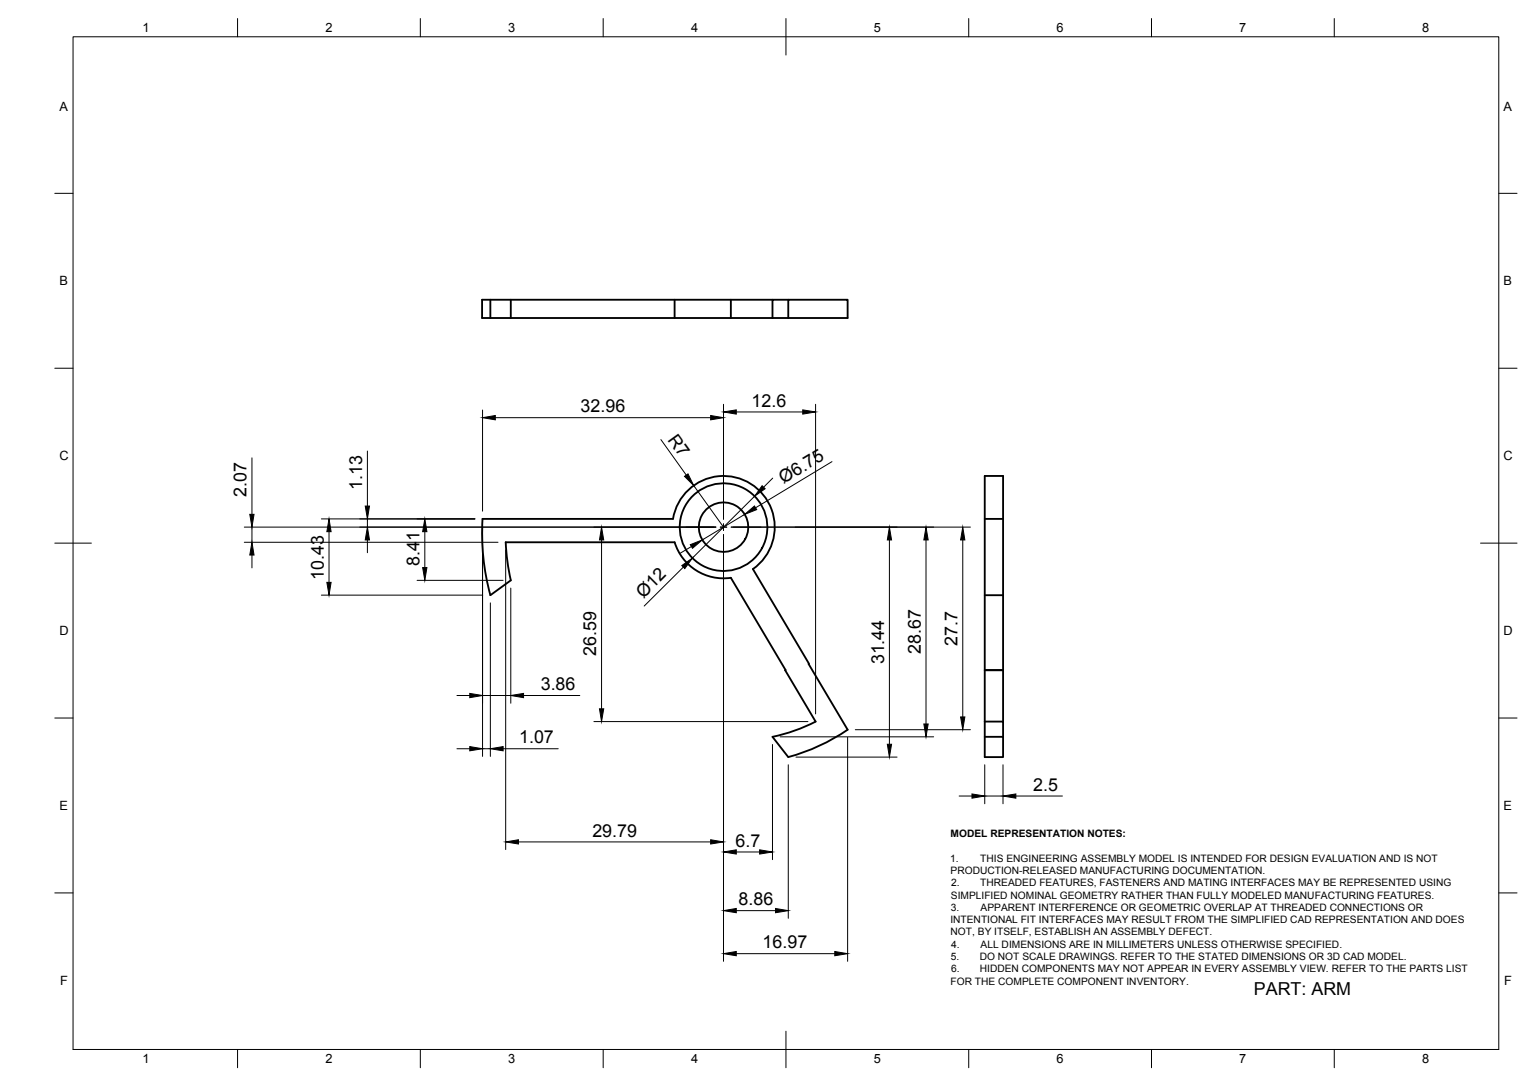
ISO-10303-21;
HEADER;
/* Generated by software containing ST-Developer
 * from STEP Tools, Inc. (www.steptools.com) 
 */

FILE_DESCRIPTION(
/* description */ (''),
/* implementation_level */ '2;1');

FILE_NAME(
/* name */ 'Arm.step',
/* time_stamp */ '2026-10-04T15:18:51-07:00',
/* author */ (''),
/* organization */ (''),
/* preprocessor_version */ 'ST-DEVELOPER v20.2',
/* originating_system */ 'Autodesk Translation Framework v15.15.0.0',
/* authorisation */ '');

FILE_SCHEMA (('AUTOMOTIVE_DESIGN { 1 0 10303 214 3 1 1 }'));
ENDSEC;

DATA;
#10=MECHANICAL_DESIGN_GEOMETRIC_PRESENTATION_REPRESENTATION('',(#77),#9891);
#58=SHAPE_REPRESENTATION_RELATIONSHIP('SRR','None',#9929,#66);
#66=ADVANCED_BREP_SHAPE_REPRESENTATION('',(#91),#9889);
#77=STYLED_ITEM('',(#9975),#91);
#91=MANIFOLD_SOLID_BREP('Body1',#5625);
#140=FACE_BOUND('',#1032,.T.);
#141=FACE_BOUND('',#1034,.T.);
#142=FACE_BOUND('',#1042,.T.);
#306=PLANE('',#6186);
#307=PLANE('',#6188);
#308=PLANE('',#6195);
#309=PLANE('',#6198);
#310=PLANE('',#6201);
#311=PLANE('',#6202);
#312=PLANE('',#6203);
#313=PLANE('',#6209);
#314=PLANE('',#6210);
#315=PLANE('',#6213);
#316=PLANE('',#6215);
#317=PLANE('',#6217);
#318=PLANE('',#6219);
#656=FACE_OUTER_BOUND('',#1030,.T.);
#657=FACE_OUTER_BOUND('',#1031,.T.);
#658=FACE_OUTER_BOUND('',#1033,.T.);
#659=FACE_OUTER_BOUND('',#1035,.T.);
#660=FACE_OUTER_BOUND('',#1036,.T.);
#661=FACE_OUTER_BOUND('',#1037,.T.);
#662=FACE_OUTER_BOUND('',#1038,.T.);
#663=FACE_OUTER_BOUND('',#1039,.T.);
#664=FACE_OUTER_BOUND('',#1040,.T.);
#665=FACE_OUTER_BOUND('',#1041,.T.);
#666=FACE_OUTER_BOUND('',#1043,.T.);
#667=FACE_OUTER_BOUND('',#1044,.T.);
#668=FACE_OUTER_BOUND('',#1045,.T.);
#669=FACE_OUTER_BOUND('',#1046,.T.);
#670=FACE_OUTER_BOUND('',#1047,.T.);
#671=FACE_OUTER_BOUND('',#1048,.T.);
#672=FACE_OUTER_BOUND('',#1049,.T.);
#673=FACE_OUTER_BOUND('',#1050,.T.);
#674=FACE_OUTER_BOUND('',#1051,.T.);
#675=FACE_OUTER_BOUND('',#1052,.T.);
#676=FACE_OUTER_BOUND('',#1053,.T.);
#1030=EDGE_LOOP('',(#4886,#4887,#4888,#4889));
#1031=EDGE_LOOP('',(#4890));
#1032=EDGE_LOOP('',(#4891));
#1033=EDGE_LOOP('',(#4892,#4893,#4894,#4895,#4896,#4897,#4898,#4899,#4900,
#4901,#4902,#4903,#4904,#4905,#4906,#4907));
#1034=EDGE_LOOP('',(#4908));
#1035=EDGE_LOOP('',(#4909,#4910,#4911,#4912));
#1036=EDGE_LOOP('',(#4913,#4914,#4915,#4916));
#1037=EDGE_LOOP('',(#4917,#4918,#4919,#4920));
#1038=EDGE_LOOP('',(#4921,#4922,#4923,#4924));
#1039=EDGE_LOOP('',(#4925,#4926,#4927,#4928));
#1040=EDGE_LOOP('',(#4929,#4930,#4931,#4932));
#1041=EDGE_LOOP('',(#4933,#4934,#4935,#4936,#4937,#4938,#4939,#4940,#4941,
#4942,#4943,#4944,#4945,#4946,#4947,#4948));
#1042=EDGE_LOOP('',(#4949));
#1043=EDGE_LOOP('',(#4950,#4951,#4952,#4953));
#1044=EDGE_LOOP('',(#4954,#4955,#4956,#4957));
#1045=EDGE_LOOP('',(#4958,#4959,#4960,#4961));
#1046=EDGE_LOOP('',(#4962,#4963,#4964,#4965));
#1047=EDGE_LOOP('',(#4966,#4967,#4968,#4969));
#1048=EDGE_LOOP('',(#4970,#4971,#4972,#4973));
#1049=EDGE_LOOP('',(#4974,#4975,#4976,#4977));
#1050=EDGE_LOOP('',(#4978,#4979,#4980,#4981));
#1051=EDGE_LOOP('',(#4982,#4983,#4984,#4985));
#1052=EDGE_LOOP('',(#4986,#4987,#4988,#4989));
#1053=EDGE_LOOP('',(#4990,#4991,#4992,#4993));
#1536=LINE('',#9530,#2000);
#1537=LINE('',#9538,#2001);
#1538=LINE('',#9540,#2002);
#1539=LINE('',#9542,#2003);
#1540=LINE('',#9546,#2004);
#1541=LINE('',#9550,#2005);
#1542=LINE('',#9554,#2006);
#1543=LINE('',#9558,#2007);
#1544=LINE('',#9560,#2008);
#1545=LINE('',#9562,#2009);
#1546=LINE('',#9566,#2010);
#1547=LINE('',#9570,#2011);
#1548=LINE('',#9572,#2012);
#1549=LINE('',#9573,#2013);
#1550=LINE('',#9578,#2014);
#1551=LINE('',#9579,#2015);
#1552=LINE('',#9582,#2016);
#1553=LINE('',#9583,#2017);
#1554=LINE('',#9587,#2018);
#1555=LINE('',#9590,#2019);
#1556=LINE('',#9591,#2020);
#1557=LINE('',#9593,#2021);
#1558=LINE('',#9596,#2022);
#1559=LINE('',#9598,#2023);
#1560=LINE('',#9602,#2024);
#1561=LINE('',#9606,#2025);
#1562=LINE('',#9610,#2026);
#1563=LINE('',#9613,#2027);
#1564=LINE('',#9617,#2028);
#1565=LINE('',#9619,#2029);
#1566=LINE('',#9621,#2030);
#1567=LINE('',#9623,#2031);
#1568=LINE('',#9625,#2032);
#1569=LINE('',#9627,#2033);
#1570=LINE('',#9629,#2034);
#1571=LINE('',#9631,#2035);
#1572=LINE('',#9633,#2036);
#1573=LINE('',#9635,#2037);
#2000=VECTOR('',#7707,3.37715398312954);
#2001=VECTOR('',#7716,10.);
#2002=VECTOR('',#7717,10.);
#2003=VECTOR('',#7718,10.);
#2004=VECTOR('',#7721,10.);
#2005=VECTOR('',#7724,10.);
#2006=VECTOR('',#7727,10.);
#2007=VECTOR('',#7730,10.);
#2008=VECTOR('',#7731,10.);
#2009=VECTOR('',#7732,10.);
#2010=VECTOR('',#7735,10.);
#2011=VECTOR('',#7740,10.);
#2012=VECTOR('',#7741,10.);
#2013=VECTOR('',#7742,9.99999999999999);
#2014=VECTOR('',#7747,10.);
#2015=VECTOR('',#7748,10.);
#2016=VECTOR('',#7751,10.);
#2017=VECTOR('',#7752,10.);
#2018=VECTOR('',#7757,10.);
#2019=VECTOR('',#7760,10.);
#2020=VECTOR('',#7761,10.);
#2021=VECTOR('',#7764,10.);
#2022=VECTOR('',#7767,9.99999999999999);
#2023=VECTOR('',#7768,10.);
#2024=VECTOR('',#7771,10.);
#2025=VECTOR('',#7774,10.);
#2026=VECTOR('',#7777,10.);
#2027=VECTOR('',#7780,10.);
#2028=VECTOR('',#7785,10.);
#2029=VECTOR('',#7788,10.);
#2030=VECTOR('',#7791,6.00000000000001);
#2031=VECTOR('',#7794,10.);
#2032=VECTOR('',#7797,10.);
#2033=VECTOR('',#7800,10.);
#2034=VECTOR('',#7803,10.);
#2035=VECTOR('',#7806,10.);
#2036=VECTOR('',#7809,10.);
#2037=VECTOR('',#7812,10.);
#2267=CIRCLE('',#6184,3.37715398312954);
#2268=CIRCLE('',#6185,3.37715398312954);
#2269=CIRCLE('',#6187,6.00000000000001);
#2270=CIRCLE('',#6189,7.00000000000001);
#2271=CIRCLE('',#6190,29.0155772121002);
#2272=CIRCLE('',#6191,32.2155772121002);
#2273=CIRCLE('',#6192,7.00000000000001);
#2274=CIRCLE('',#6193,26.714151341222);
#2275=CIRCLE('',#6194,23.514151341222);
#2276=CIRCLE('',#6197,26.714151341222);
#2277=CIRCLE('',#6200,23.514151341222);
#2278=CIRCLE('',#6204,7.00000000000001);
#2279=CIRCLE('',#6205,32.2155772121003);
#2280=CIRCLE('',#6206,29.0155772121003);
#2281=CIRCLE('',#6207,7.00000000000001);
#2282=CIRCLE('',#6208,6.00000000000001);
#2770=VERTEX_POINT('',#9527);
#2771=VERTEX_POINT('',#9529);
#2772=VERTEX_POINT('',#9533);
#2773=VERTEX_POINT('',#9536);
#2774=VERTEX_POINT('',#9537);
#2775=VERTEX_POINT('',#9539);
#2776=VERTEX_POINT('',#9541);
#2777=VERTEX_POINT('',#9543);
#2778=VERTEX_POINT('',#9545);
#2779=VERTEX_POINT('',#9547);
#2780=VERTEX_POINT('',#9549);
#2781=VERTEX_POINT('',#9551);
#2782=VERTEX_POINT('',#9553);
#2783=VERTEX_POINT('',#9555);
#2784=VERTEX_POINT('',#9557);
#2785=VERTEX_POINT('',#9559);
#2786=VERTEX_POINT('',#9561);
#2787=VERTEX_POINT('',#9563);
#2788=VERTEX_POINT('',#9565);
#2789=VERTEX_POINT('',#9569);
#2790=VERTEX_POINT('',#9571);
#2791=VERTEX_POINT('',#9575);
#2792=VERTEX_POINT('',#9576);
#2793=VERTEX_POINT('',#9581);
#2794=VERTEX_POINT('',#9585);
#2795=VERTEX_POINT('',#9589);
#2796=VERTEX_POINT('',#9595);
#2797=VERTEX_POINT('',#9597);
#2798=VERTEX_POINT('',#9599);
#2799=VERTEX_POINT('',#9601);
#2800=VERTEX_POINT('',#9603);
#2801=VERTEX_POINT('',#9605);
#2802=VERTEX_POINT('',#9607);
#2803=VERTEX_POINT('',#9609);
#2804=VERTEX_POINT('',#9611);
#2805=VERTEX_POINT('',#9614);
#3488=EDGE_CURVE('',#2770,#2770,#2267,.F.);
#3489=EDGE_CURVE('',#2770,#2771,#1536,.T.);
#3490=EDGE_CURVE('',#2771,#2771,#2268,.T.);
#3491=EDGE_CURVE('',#2772,#2772,#2269,.T.);
#3492=EDGE_CURVE('',#2773,#2774,#1537,.T.);
#3493=EDGE_CURVE('',#2774,#2775,#1538,.T.);
#3494=EDGE_CURVE('',#2775,#2776,#1539,.T.);
#3495=EDGE_CURVE('',#2776,#2777,#2270,.T.);
#3496=EDGE_CURVE('',#2777,#2778,#1540,.T.);
#3497=EDGE_CURVE('',#2778,#2779,#2271,.T.);
#3498=EDGE_CURVE('',#2779,#2780,#1541,.T.);
#3499=EDGE_CURVE('',#2780,#2781,#2272,.T.);
#3500=EDGE_CURVE('',#2781,#2782,#1542,.T.);
#3501=EDGE_CURVE('',#2782,#2783,#2273,.T.);
#3502=EDGE_CURVE('',#2783,#2784,#1543,.T.);
#3503=EDGE_CURVE('',#2784,#2785,#1544,.T.);
#3504=EDGE_CURVE('',#2785,#2786,#1545,.T.);
#3505=EDGE_CURVE('',#2786,#2787,#2274,.T.);
#3506=EDGE_CURVE('',#2787,#2788,#1546,.T.);
#3507=EDGE_CURVE('',#2788,#2773,#2275,.T.);
#3508=EDGE_CURVE('',#2775,#2789,#1547,.T.);
#3509=EDGE_CURVE('',#2774,#2790,#1548,.T.);
#3510=EDGE_CURVE('',#2790,#2789,#1549,.T.);
#3511=EDGE_CURVE('',#2791,#2792,#2276,.T.);
#3512=EDGE_CURVE('',#2792,#2787,#1550,.T.);
#3513=EDGE_CURVE('',#2791,#2786,#1551,.T.);
#3514=EDGE_CURVE('',#2792,#2793,#1552,.T.);
#3515=EDGE_CURVE('',#2793,#2788,#1553,.T.);
#3516=EDGE_CURVE('',#2794,#2793,#2277,.T.);
#3517=EDGE_CURVE('',#2794,#2773,#1554,.T.);
#3518=EDGE_CURVE('',#2795,#2785,#1555,.T.);
#3519=EDGE_CURVE('',#2791,#2795,#1556,.T.);
#3520=EDGE_CURVE('',#2794,#2790,#1557,.T.);
#3521=EDGE_CURVE('',#2795,#2796,#1558,.T.);
#3522=EDGE_CURVE('',#2796,#2797,#1559,.T.);
#3523=EDGE_CURVE('',#2798,#2797,#2278,.T.);
#3524=EDGE_CURVE('',#2798,#2799,#1560,.T.);
#3525=EDGE_CURVE('',#2800,#2799,#2279,.T.);
#3526=EDGE_CURVE('',#2801,#2800,#1561,.T.);
#3527=EDGE_CURVE('',#2801,#2802,#2280,.T.);
#3528=EDGE_CURVE('',#2803,#2802,#1562,.T.);
#3529=EDGE_CURVE('',#2804,#2803,#2281,.T.);
#3530=EDGE_CURVE('',#2789,#2804,#1563,.T.);
#3531=EDGE_CURVE('',#2805,#2805,#2282,.T.);
#3532=EDGE_CURVE('',#2796,#2784,#1564,.T.);
#3533=EDGE_CURVE('',#2797,#2783,#1565,.T.);
#3534=EDGE_CURVE('',#2805,#2772,#1566,.T.);
#3535=EDGE_CURVE('',#2798,#2782,#1567,.T.);
#3536=EDGE_CURVE('',#2799,#2781,#1568,.T.);
#3537=EDGE_CURVE('',#2800,#2780,#1569,.T.);
#3538=EDGE_CURVE('',#2801,#2779,#1570,.T.);
#3539=EDGE_CURVE('',#2802,#2778,#1571,.T.);
#3540=EDGE_CURVE('',#2803,#2777,#1572,.T.);
#3541=EDGE_CURVE('',#2804,#2776,#1573,.T.);
#4886=ORIENTED_EDGE('',*,*,#3488,.F.);
#4887=ORIENTED_EDGE('',*,*,#3489,.T.);
#4888=ORIENTED_EDGE('',*,*,#3490,.F.);
#4889=ORIENTED_EDGE('',*,*,#3489,.F.);
#4890=ORIENTED_EDGE('',*,*,#3491,.T.);
#4891=ORIENTED_EDGE('',*,*,#3488,.T.);
#4892=ORIENTED_EDGE('',*,*,#3492,.T.);
#4893=ORIENTED_EDGE('',*,*,#3493,.T.);
#4894=ORIENTED_EDGE('',*,*,#3494,.T.);
#4895=ORIENTED_EDGE('',*,*,#3495,.T.);
#4896=ORIENTED_EDGE('',*,*,#3496,.T.);
#4897=ORIENTED_EDGE('',*,*,#3497,.T.);
#4898=ORIENTED_EDGE('',*,*,#3498,.T.);
#4899=ORIENTED_EDGE('',*,*,#3499,.T.);
#4900=ORIENTED_EDGE('',*,*,#3500,.T.);
#4901=ORIENTED_EDGE('',*,*,#3501,.T.);
#4902=ORIENTED_EDGE('',*,*,#3502,.T.);
#4903=ORIENTED_EDGE('',*,*,#3503,.T.);
#4904=ORIENTED_EDGE('',*,*,#3504,.T.);
#4905=ORIENTED_EDGE('',*,*,#3505,.T.);
#4906=ORIENTED_EDGE('',*,*,#3506,.T.);
#4907=ORIENTED_EDGE('',*,*,#3507,.T.);
#4908=ORIENTED_EDGE('',*,*,#3490,.T.);
#4909=ORIENTED_EDGE('',*,*,#3508,.F.);
#4910=ORIENTED_EDGE('',*,*,#3493,.F.);
#4911=ORIENTED_EDGE('',*,*,#3509,.T.);
#4912=ORIENTED_EDGE('',*,*,#3510,.T.);
#4913=ORIENTED_EDGE('',*,*,#3511,.T.);
#4914=ORIENTED_EDGE('',*,*,#3512,.T.);
#4915=ORIENTED_EDGE('',*,*,#3505,.F.);
#4916=ORIENTED_EDGE('',*,*,#3513,.F.);
#4917=ORIENTED_EDGE('',*,*,#3514,.T.);
#4918=ORIENTED_EDGE('',*,*,#3515,.T.);
#4919=ORIENTED_EDGE('',*,*,#3506,.F.);
#4920=ORIENTED_EDGE('',*,*,#3512,.F.);
#4921=ORIENTED_EDGE('',*,*,#3516,.F.);
#4922=ORIENTED_EDGE('',*,*,#3517,.T.);
#4923=ORIENTED_EDGE('',*,*,#3507,.F.);
#4924=ORIENTED_EDGE('',*,*,#3515,.F.);
#4925=ORIENTED_EDGE('',*,*,#3518,.F.);
#4926=ORIENTED_EDGE('',*,*,#3519,.F.);
#4927=ORIENTED_EDGE('',*,*,#3513,.T.);
#4928=ORIENTED_EDGE('',*,*,#3504,.F.);
#4929=ORIENTED_EDGE('',*,*,#3509,.F.);
#4930=ORIENTED_EDGE('',*,*,#3492,.F.);
#4931=ORIENTED_EDGE('',*,*,#3517,.F.);
#4932=ORIENTED_EDGE('',*,*,#3520,.T.);
#4933=ORIENTED_EDGE('',*,*,#3510,.F.);
#4934=ORIENTED_EDGE('',*,*,#3520,.F.);
#4935=ORIENTED_EDGE('',*,*,#3516,.T.);
#4936=ORIENTED_EDGE('',*,*,#3514,.F.);
#4937=ORIENTED_EDGE('',*,*,#3511,.F.);
#4938=ORIENTED_EDGE('',*,*,#3519,.T.);
#4939=ORIENTED_EDGE('',*,*,#3521,.T.);
#4940=ORIENTED_EDGE('',*,*,#3522,.T.);
#4941=ORIENTED_EDGE('',*,*,#3523,.F.);
#4942=ORIENTED_EDGE('',*,*,#3524,.T.);
#4943=ORIENTED_EDGE('',*,*,#3525,.F.);
#4944=ORIENTED_EDGE('',*,*,#3526,.F.);
#4945=ORIENTED_EDGE('',*,*,#3527,.T.);
#4946=ORIENTED_EDGE('',*,*,#3528,.F.);
#4947=ORIENTED_EDGE('',*,*,#3529,.F.);
#4948=ORIENTED_EDGE('',*,*,#3530,.F.);
#4949=ORIENTED_EDGE('',*,*,#3531,.F.);
#4950=ORIENTED_EDGE('',*,*,#3518,.T.);
#4951=ORIENTED_EDGE('',*,*,#3503,.F.);
#4952=ORIENTED_EDGE('',*,*,#3532,.F.);
#4953=ORIENTED_EDGE('',*,*,#3521,.F.);
#4954=ORIENTED_EDGE('',*,*,#3532,.T.);
#4955=ORIENTED_EDGE('',*,*,#3502,.F.);
#4956=ORIENTED_EDGE('',*,*,#3533,.F.);
#4957=ORIENTED_EDGE('',*,*,#3522,.F.);
#4958=ORIENTED_EDGE('',*,*,#3531,.T.);
#4959=ORIENTED_EDGE('',*,*,#3534,.T.);
#4960=ORIENTED_EDGE('',*,*,#3491,.F.);
#4961=ORIENTED_EDGE('',*,*,#3534,.F.);
#4962=ORIENTED_EDGE('',*,*,#3523,.T.);
#4963=ORIENTED_EDGE('',*,*,#3533,.T.);
#4964=ORIENTED_EDGE('',*,*,#3501,.F.);
#4965=ORIENTED_EDGE('',*,*,#3535,.F.);
#4966=ORIENTED_EDGE('',*,*,#3524,.F.);
#4967=ORIENTED_EDGE('',*,*,#3535,.T.);
#4968=ORIENTED_EDGE('',*,*,#3500,.F.);
#4969=ORIENTED_EDGE('',*,*,#3536,.F.);
#4970=ORIENTED_EDGE('',*,*,#3525,.T.);
#4971=ORIENTED_EDGE('',*,*,#3536,.T.);
#4972=ORIENTED_EDGE('',*,*,#3499,.F.);
#4973=ORIENTED_EDGE('',*,*,#3537,.F.);
#4974=ORIENTED_EDGE('',*,*,#3526,.T.);
#4975=ORIENTED_EDGE('',*,*,#3537,.T.);
#4976=ORIENTED_EDGE('',*,*,#3498,.F.);
#4977=ORIENTED_EDGE('',*,*,#3538,.F.);
#4978=ORIENTED_EDGE('',*,*,#3527,.F.);
#4979=ORIENTED_EDGE('',*,*,#3538,.T.);
#4980=ORIENTED_EDGE('',*,*,#3497,.F.);
#4981=ORIENTED_EDGE('',*,*,#3539,.F.);
#4982=ORIENTED_EDGE('',*,*,#3528,.T.);
#4983=ORIENTED_EDGE('',*,*,#3539,.T.);
#4984=ORIENTED_EDGE('',*,*,#3496,.F.);
#4985=ORIENTED_EDGE('',*,*,#3540,.F.);
#4986=ORIENTED_EDGE('',*,*,#3529,.T.);
#4987=ORIENTED_EDGE('',*,*,#3540,.T.);
#4988=ORIENTED_EDGE('',*,*,#3495,.F.);
#4989=ORIENTED_EDGE('',*,*,#3541,.F.);
#4990=ORIENTED_EDGE('',*,*,#3508,.T.);
#4991=ORIENTED_EDGE('',*,*,#3530,.T.);
#4992=ORIENTED_EDGE('',*,*,#3541,.T.);
#4993=ORIENTED_EDGE('',*,*,#3494,.F.);
#5268=CYLINDRICAL_SURFACE('',#6183,3.37715398312954);
#5269=CYLINDRICAL_SURFACE('',#6196,26.714151341222);
#5270=CYLINDRICAL_SURFACE('',#6199,23.514151341222);
#5271=CYLINDRICAL_SURFACE('',#6211,6.00000000000001);
#5272=CYLINDRICAL_SURFACE('',#6212,7.00000000000001);
#5273=CYLINDRICAL_SURFACE('',#6214,32.2155772121003);
#5274=CYLINDRICAL_SURFACE('',#6216,29.0155772121003);
#5275=CYLINDRICAL_SURFACE('',#6218,7.00000000000001);
#5535=ADVANCED_FACE('',(#656),#5268,.F.);
#5536=ADVANCED_FACE('',(#657,#140),#306,.F.);
#5537=ADVANCED_FACE('',(#658,#141),#307,.T.);
#5538=ADVANCED_FACE('',(#659),#308,.T.);
#5539=ADVANCED_FACE('',(#660),#5269,.T.);
#5540=ADVANCED_FACE('',(#661),#309,.T.);
#5541=ADVANCED_FACE('',(#662),#5270,.F.);
#5542=ADVANCED_FACE('',(#663),#310,.T.);
#5543=ADVANCED_FACE('',(#664),#311,.T.);
#5544=ADVANCED_FACE('',(#665,#142),#312,.F.);
#5545=ADVANCED_FACE('',(#666),#313,.F.);
#5546=ADVANCED_FACE('',(#667),#314,.T.);
#5547=ADVANCED_FACE('',(#668),#5271,.F.);
#5548=ADVANCED_FACE('',(#669),#5272,.T.);
#5549=ADVANCED_FACE('',(#670),#315,.T.);
#5550=ADVANCED_FACE('',(#671),#5273,.T.);
#5551=ADVANCED_FACE('',(#672),#316,.T.);
#5552=ADVANCED_FACE('',(#673),#5274,.F.);
#5553=ADVANCED_FACE('',(#674),#317,.T.);
#5554=ADVANCED_FACE('',(#675),#5275,.T.);
#5555=ADVANCED_FACE('',(#676),#318,.T.);
#5625=CLOSED_SHELL('',(#5535,#5536,#5537,#5538,#5539,#5540,#5541,#5542,
#5543,#5544,#5545,#5546,#5547,#5548,#5549,#5550,#5551,#5552,#5553,#5554,
#5555));
#6182=AXIS2_PLACEMENT_3D('',#9525,#7701,#7702);
#6183=AXIS2_PLACEMENT_3D('',#9526,#7703,#7704);
#6184=AXIS2_PLACEMENT_3D('',#9528,#7705,#7706);
#6185=AXIS2_PLACEMENT_3D('',#9531,#7708,#7709);
#6186=AXIS2_PLACEMENT_3D('',#9532,#7710,#7711);
#6187=AXIS2_PLACEMENT_3D('',#9534,#7712,#7713);
#6188=AXIS2_PLACEMENT_3D('',#9535,#7714,#7715);
#6189=AXIS2_PLACEMENT_3D('',#9544,#7719,#7720);
#6190=AXIS2_PLACEMENT_3D('',#9548,#7722,#7723);
#6191=AXIS2_PLACEMENT_3D('',#9552,#7725,#7726);
#6192=AXIS2_PLACEMENT_3D('',#9556,#7728,#7729);
#6193=AXIS2_PLACEMENT_3D('',#9564,#7733,#7734);
#6194=AXIS2_PLACEMENT_3D('',#9567,#7736,#7737);
#6195=AXIS2_PLACEMENT_3D('',#9568,#7738,#7739);
#6196=AXIS2_PLACEMENT_3D('',#9574,#7743,#7744);
#6197=AXIS2_PLACEMENT_3D('',#9577,#7745,#7746);
#6198=AXIS2_PLACEMENT_3D('',#9580,#7749,#7750);
#6199=AXIS2_PLACEMENT_3D('',#9584,#7753,#7754);
#6200=AXIS2_PLACEMENT_3D('',#9586,#7755,#7756);
#6201=AXIS2_PLACEMENT_3D('',#9588,#7758,#7759);
#6202=AXIS2_PLACEMENT_3D('',#9592,#7762,#7763);
#6203=AXIS2_PLACEMENT_3D('',#9594,#7765,#7766);
#6204=AXIS2_PLACEMENT_3D('',#9600,#7769,#7770);
#6205=AXIS2_PLACEMENT_3D('',#9604,#7772,#7773);
#6206=AXIS2_PLACEMENT_3D('',#9608,#7775,#7776);
#6207=AXIS2_PLACEMENT_3D('',#9612,#7778,#7779);
#6208=AXIS2_PLACEMENT_3D('',#9615,#7781,#7782);
#6209=AXIS2_PLACEMENT_3D('',#9616,#7783,#7784);
#6210=AXIS2_PLACEMENT_3D('',#9618,#7786,#7787);
#6211=AXIS2_PLACEMENT_3D('',#9620,#7789,#7790);
#6212=AXIS2_PLACEMENT_3D('',#9622,#7792,#7793);
#6213=AXIS2_PLACEMENT_3D('',#9624,#7795,#7796);
#6214=AXIS2_PLACEMENT_3D('',#9626,#7798,#7799);
#6215=AXIS2_PLACEMENT_3D('',#9628,#7801,#7802);
#6216=AXIS2_PLACEMENT_3D('',#9630,#7804,#7805);
#6217=AXIS2_PLACEMENT_3D('',#9632,#7807,#7808);
#6218=AXIS2_PLACEMENT_3D('',#9634,#7810,#7811);
#6219=AXIS2_PLACEMENT_3D('',#9636,#7813,#7814);
#7701=DIRECTION('axis',(0.,0.,1.));
#7702=DIRECTION('refdir',(1.,0.,0.));
#7703=DIRECTION('center_axis',(0.,-1.,0.));
#7704=DIRECTION('ref_axis',(1.,0.,0.));
#7705=DIRECTION('center_axis',(0.,1.,0.));
#7706=DIRECTION('ref_axis',(1.,0.,0.));
#7707=DIRECTION('',(0.,-1.,0.));
#7708=DIRECTION('center_axis',(0.,1.,0.));
#7709=DIRECTION('ref_axis',(1.,0.,0.));
#7710=DIRECTION('center_axis',(0.,-1.,0.));
#7711=DIRECTION('ref_axis',(1.,0.,0.));
#7712=DIRECTION('center_axis',(0.,1.,0.));
#7713=DIRECTION('ref_axis',(1.,0.,0.));
#7714=DIRECTION('center_axis',(0.,-1.,0.));
#7715=DIRECTION('ref_axis',(1.,0.,0.));
#7716=DIRECTION('',(0.860147585785704,0.,0.510045224139021));
#7717=DIRECTION('',(-0.510045224139015,0.,0.860147585785708));
#7718=DIRECTION('',(0.860147585785706,0.,0.510045224139018));
#7719=DIRECTION('center_axis',(0.,-1.,0.));
#7720=DIRECTION('ref_axis',(-0.600758197939069,0.,-0.799430789755438));
#7721=DIRECTION('',(0.877406199933791,0.,-0.479748225966229));
#7722=DIRECTION('center_axis',(0.,1.,0.));
#7723=DIRECTION('ref_axis',(0.749053332236673,0.,-0.662509702166796));
#7724=DIRECTION('',(0.429092562599351,0.,-0.903260523172535));
#7725=DIRECTION('center_axis',(0.,-1.,0.));
#7726=DIRECTION('ref_axis',(0.72057468488707,0.,-0.693377331256149));
#7727=DIRECTION('',(-0.877406199933791,0.,0.479748225966229));
#7728=DIRECTION('center_axis',(0.,-1.,0.));
#7729=DIRECTION('ref_axis',(0.943439642400352,0.,-0.331544327575508));
#7730=DIRECTION('',(-0.860147585785706,0.,-0.510045224139018));
#7731=DIRECTION('',(0.510045224139015,0.,-0.860147585785708));
#7732=DIRECTION('',(-0.860147585785706,0.,-0.510045224139018));
#7733=DIRECTION('center_axis',(0.,-1.,0.));
#7734=DIRECTION('ref_axis',(-0.891523131063977,0.,-0.452975172363656));
#7735=DIRECTION('',(0.91803072008761,0.,0.39650926467792));
#7736=DIRECTION('center_axis',(0.,1.,0.));
#7737=DIRECTION('ref_axis',(-0.826791968384381,0.,-0.562507814181351));
#7738=DIRECTION('center_axis',(0.860147585785706,0.,0.510045224139019));
#7739=DIRECTION('ref_axis',(0.510045224139019,0.,-0.860147585785706));
#7740=DIRECTION('',(0.,1.,0.));
#7741=DIRECTION('',(0.,1.,0.));
#7742=DIRECTION('',(-0.510045224139019,0.,0.860147585785705));
#7743=DIRECTION('center_axis',(0.,-1.,0.));
#7744=DIRECTION('ref_axis',(-0.891523131063977,0.,-0.452975172363656));
#7745=DIRECTION('center_axis',(0.,-1.,0.));
#7746=DIRECTION('ref_axis',(-0.891523131063977,0.,-0.452975172363656));
#7747=DIRECTION('',(0.,-1.,0.));
#7748=DIRECTION('',(0.,-1.,0.));
#7749=DIRECTION('center_axis',(0.396509264677948,0.,-0.918030720087598));
#7750=DIRECTION('ref_axis',(0.918030720087598,0.,0.396509264677948));
#7751=DIRECTION('',(0.918030720087598,0.,0.396509264677948));
#7752=DIRECTION('',(0.,-1.,0.));
#7753=DIRECTION('center_axis',(0.,-1.,0.));
#7754=DIRECTION('ref_axis',(-0.893553614971487,0.,-0.448956498083487));
#7755=DIRECTION('center_axis',(0.,-1.,0.));
#7756=DIRECTION('ref_axis',(-0.893553614971487,0.,-0.448956498083487));
#7757=DIRECTION('',(0.,-1.,0.));
#7758=DIRECTION('center_axis',(-0.510045224139018,0.,0.860147585785706));
#7759=DIRECTION('ref_axis',(-0.860147585785706,0.,-0.510045224139018));
#7760=DIRECTION('',(0.,-1.,0.));
#7761=DIRECTION('',(0.860147585785706,0.,0.510045224139018));
#7762=DIRECTION('center_axis',(0.510045224139018,0.,-0.860147585785706));
#7763=DIRECTION('ref_axis',(0.860147585785706,0.,0.510045224139018));
#7764=DIRECTION('',(0.860147585785706,0.,0.510045224139018));
#7765=DIRECTION('center_axis',(0.,-1.,0.));
#7766=DIRECTION('ref_axis',(1.,0.,0.));
#7767=DIRECTION('',(-0.510045224139019,0.,0.860147585785705));
#7768=DIRECTION('',(0.860147585785706,0.,0.510045224139018));
#7769=DIRECTION('center_axis',(0.,-1.,0.));
#7770=DIRECTION('ref_axis',(1.,0.,0.));
#7771=DIRECTION('',(0.877406199933791,0.,-0.479748225966229));
#7772=DIRECTION('center_axis',(0.,-1.,0.));
#7773=DIRECTION('ref_axis',(0.720574684887071,0.,-0.693377331256149));
#7774=DIRECTION('',(0.429092562599351,0.,-0.903260523172535));
#7775=DIRECTION('center_axis',(0.,-1.,0.));
#7776=DIRECTION('ref_axis',(0.749053332236673,0.,-0.662509702166795));
#7777=DIRECTION('',(0.877406199933792,0.,-0.479748225966228));
#7778=DIRECTION('center_axis',(0.,-1.,0.));
#7779=DIRECTION('ref_axis',(1.,0.,0.));
#7780=DIRECTION('',(0.860147585785706,0.,0.510045224139018));
#7781=DIRECTION('center_axis',(0.,1.,0.));
#7782=DIRECTION('ref_axis',(1.,0.,0.));
#7783=DIRECTION('center_axis',(0.860147585785706,0.,0.510045224139019));
#7784=DIRECTION('ref_axis',(0.510045224139019,0.,-0.860147585785706));
#7785=DIRECTION('',(0.,-1.,0.));
#7786=DIRECTION('center_axis',(-0.510045224139018,0.,0.860147585785706));
#7787=DIRECTION('ref_axis',(-0.860147585785706,0.,-0.510045224139018));
#7788=DIRECTION('',(0.,-1.,0.));
#7789=DIRECTION('center_axis',(0.,-1.,0.));
#7790=DIRECTION('ref_axis',(1.,0.,0.));
#7791=DIRECTION('',(0.,-1.,0.));
#7792=DIRECTION('center_axis',(0.,-1.,0.));
#7793=DIRECTION('ref_axis',(-0.0606108082303955,0.,0.998161474875512));
#7794=DIRECTION('',(0.,-1.,0.));
#7795=DIRECTION('center_axis',(0.479748225966229,0.,0.877406199933791));
#7796=DIRECTION('ref_axis',(-0.877406199933791,0.,0.479748225966229));
#7797=DIRECTION('',(0.,-1.,0.));
#7798=DIRECTION('center_axis',(0.,-1.,0.));
#7799=DIRECTION('ref_axis',(0.720574684887071,0.,-0.693377331256149));
#7800=DIRECTION('',(0.,-1.,0.));
#7801=DIRECTION('center_axis',(-0.903260523172535,0.,-0.429092562599351));
#7802=DIRECTION('ref_axis',(0.429092562599351,0.,-0.903260523172535));
#7803=DIRECTION('',(0.,-1.,0.));
#7804=DIRECTION('center_axis',(0.,-1.,0.));
#7805=DIRECTION('ref_axis',(0.749053332236673,0.,-0.662509702166795));
#7806=DIRECTION('',(0.,-1.,0.));
#7807=DIRECTION('center_axis',(-0.479748225966228,0.,-0.877406199933792));
#7808=DIRECTION('ref_axis',(0.877406199933792,0.,-0.479748225966228));
#7809=DIRECTION('',(0.,-1.,0.));
#7810=DIRECTION('center_axis',(0.,-1.,0.));
#7811=DIRECTION('ref_axis',(1.,0.,0.));
#7812=DIRECTION('',(0.,-1.,0.));
#7813=DIRECTION('center_axis',(0.510045224139018,0.,-0.860147585785706));
#7814=DIRECTION('ref_axis',(0.860147585785706,0.,0.510045224139018));
#9525=CARTESIAN_POINT('',(0.,0.,0.));
#9526=CARTESIAN_POINT('Origin',(3.64981768126446E-16,-4.,86.8));
#9527=CARTESIAN_POINT('',(-3.37715398312954,-4.,86.8));
#9528=CARTESIAN_POINT('Origin',(3.64981768126446E-16,-4.,86.8));
#9529=CARTESIAN_POINT('',(-3.37715398312954,-4.5,86.8));
#9530=CARTESIAN_POINT('',(-3.37715398312954,-4.,86.8));
#9531=CARTESIAN_POINT('Origin',(3.64981768126446E-16,-4.5,86.8));
#9532=CARTESIAN_POINT('Origin',(0.637540569301853,-4.,78.5706101655767));
#9533=CARTESIAN_POINT('',(-6.00000000000001,-4.,86.8));
#9534=CARTESIAN_POINT('Origin',(5.11429163215176E-16,-4.,86.8));
#9535=CARTESIAN_POINT('Origin',(0.637540569301853,-4.5,78.5706101655767));
#9536=CARTESIAN_POINT('',(-23.8080041831819,-4.5,69.5119859113367));
#9537=CARTESIAN_POINT('',(-16.7912595803416,-4.5,73.6727335932742));
#9538=CARTESIAN_POINT('',(-23.8080041831819,-4.5,69.5119859113367));
#9539=CARTESIAN_POINT('',(-16.8211392806367,-4.5,73.7231231486636));
#9540=CARTESIAN_POINT('',(-16.7912595803416,-4.5,73.6727335932742));
#9541=CARTESIAN_POINT('',(-4.20530738557349,-4.5,81.2039844717119));
#9542=CARTESIAN_POINT('',(-16.8211392806367,-4.5,73.7231231486636));
#9543=CARTESIAN_POINT('',(4.87558269014984,-4.5,81.777182719677));
#9544=CARTESIAN_POINT('Origin',(5.11429163215176E-16,-4.5,86.8));
#9545=CARTESIAN_POINT('',(25.14540508495,-4.5,70.6940477528968));
#9546=CARTESIAN_POINT('',(4.87558269014983,-4.5,81.777182719677));
#9547=CARTESIAN_POINT('',(22.0328538621538,-4.5,66.4556698663697));
#9548=CARTESIAN_POINT('Origin',(0.298639064659696,-4.5,85.6787712833559));
#9549=CARTESIAN_POINT('',(23.5123684627238,-4.5,63.3412203311535));
#9550=CARTESIAN_POINT('',(22.0328538621538,-4.5,66.4556698663697));
#9551=CARTESIAN_POINT('',(29.4580576969316,-4.5,71.983088746998));
#9552=CARTESIAN_POINT('Origin',(0.298639064659696,-4.5,85.6787712833559));
#9553=CARTESIAN_POINT('',(6.60407749680247,-4.5,84.4791897069714));
#9554=CARTESIAN_POINT('',(29.4580576969316,-4.5,71.983088746998));
#9555=CARTESIAN_POINT('',(-6.27473995448561,-4.5,83.6971563842852));
#9556=CARTESIAN_POINT('Origin',(5.11429163215176E-16,-4.5,86.8));
#9557=CARTESIAN_POINT('',(-19.225775115544,-4.5,76.0175282126611));
#9558=CARTESIAN_POINT('',(-6.27473995448561,-4.5,83.6971563842852));
#9559=CARTESIAN_POINT('',(-19.1958954152489,-4.5,75.9671386572717));
#9560=CARTESIAN_POINT('',(-19.225775115544,-4.5,76.0175282126611));
#9561=CARTESIAN_POINT('',(-28.1829765583279,-4.5,70.6380324762781));
#9562=CARTESIAN_POINT('',(-19.1958954152489,-4.5,75.9671386572717));
#9563=CARTESIAN_POINT('',(-22.8617076926603,-4.5,63.4624614786761));
#9564=CARTESIAN_POINT('Origin',(-4.36669271088479,-4.5,82.738879784617));
#9565=CARTESIAN_POINT('',(-19.6350203672456,-4.5,64.8561091973757));
#9566=CARTESIAN_POINT('',(-22.8617076926603,-4.5,63.4624614786761));
#9567=CARTESIAN_POINT('Origin',(-4.36669271088479,-4.5,82.738879784617));
#9568=CARTESIAN_POINT('Origin',(-18.4234042975864,-2.,76.4252058677884));
#9569=CARTESIAN_POINT('',(-16.8211392806367,-2.,73.7231231486636));
#9570=CARTESIAN_POINT('',(-16.8211392806367,-2.,73.7231231486636));
#9571=CARTESIAN_POINT('',(-16.7912595803416,-2.,73.6727335932742));
#9572=CARTESIAN_POINT('',(-16.7912595803416,-2.,73.6727335932742));
#9573=CARTESIAN_POINT('',(-16.4205260287817,-2.,73.0475232114257));
#9574=CARTESIAN_POINT('Origin',(-4.36669271088479,-2.,82.738879784617));
#9575=CARTESIAN_POINT('',(-28.1829765583279,-2.,70.6380324762781));
#9576=CARTESIAN_POINT('',(-22.8617076926605,-2.,63.4624614786759));
#9577=CARTESIAN_POINT('Origin',(-4.36669271088479,-2.,82.738879784617));
#9578=CARTESIAN_POINT('',(-22.8617076926605,-2.,63.4624614786759));
#9579=CARTESIAN_POINT('',(-28.1829765583279,-2.,70.6380324762781));
#9580=CARTESIAN_POINT('Origin',(-22.8617076926605,-2.,63.4624614786759));
#9581=CARTESIAN_POINT('',(-19.6350203672463,-2.,64.8561091973748));
#9582=CARTESIAN_POINT('',(-22.8617076926605,-2.,63.4624614786759));
#9583=CARTESIAN_POINT('',(-19.6350203672463,-2.,64.8561091973748));
#9584=CARTESIAN_POINT('Origin',(-4.36669271088479,-2.,82.738879784617));
#9585=CARTESIAN_POINT('',(-23.808004183182,-2.,69.5119859113367));
#9586=CARTESIAN_POINT('Origin',(-4.36669271088479,-2.,82.738879784617));
#9587=CARTESIAN_POINT('',(-23.808004183182,-2.,69.5119859113367));
#9588=CARTESIAN_POINT('Origin',(-5.47236913652802,-2.,84.1048340394125));
#9589=CARTESIAN_POINT('',(-19.1958954152489,-2.,75.9671386572717));
#9590=CARTESIAN_POINT('',(-19.1958954152489,-2.,75.9671386572717));
#9591=CARTESIAN_POINT('',(-31.1673936222204,-2.,68.8683505107269));
#9592=CARTESIAN_POINT('Origin',(-23.808004183182,-2.,69.5119859113367));
#9593=CARTESIAN_POINT('',(-29.5352489049756,-2.,66.1158782362127));
#9594=CARTESIAN_POINT('Origin',(0.236355160323063,-2.,78.4273919117743));
#9595=CARTESIAN_POINT('',(-19.225775115544,-2.,76.0175282126611));
#9596=CARTESIAN_POINT('',(-17.2228968467393,-2.,72.6398455562984));
#9597=CARTESIAN_POINT('',(-6.2747399544856,-2.,83.6971563842852));
#9598=CARTESIAN_POINT('',(-31.969764440178,-2.,68.4606728555997));
#9599=CARTESIAN_POINT('',(6.60407749680247,-2.,84.4791897069714));
#9600=CARTESIAN_POINT('Origin',(5.11429163215176E-16,-2.,86.8));
#9601=CARTESIAN_POINT('',(29.4580576969316,-2.,71.983088746998));
#9602=CARTESIAN_POINT('',(6.60407749680247,-2.,84.4791897069714));
#9603=CARTESIAN_POINT('',(23.5123684627238,-2.,63.3412203311535));
#9604=CARTESIAN_POINT('Origin',(0.29863906465954,-2.,85.678771283356));
#9605=CARTESIAN_POINT('',(22.0328538621538,-2.,66.4556698663697));
#9606=CARTESIAN_POINT('',(22.0328538621538,-2.,66.4556698663697));
#9607=CARTESIAN_POINT('',(25.14540508495,-2.,70.6940477528968));
#9608=CARTESIAN_POINT('Origin',(0.29863906465954,-2.,85.678771283356));
#9609=CARTESIAN_POINT('',(4.87558269014984,-2.,81.777182719677));
#9610=CARTESIAN_POINT('',(4.87558269014984,-2.,81.777182719677));
#9611=CARTESIAN_POINT('',(-4.20530738557349,-2.,81.2039844717119));
#9612=CARTESIAN_POINT('Origin',(5.11429163215176E-16,-2.,86.8));
#9613=CARTESIAN_POINT('',(-30.3376197229332,-2.,65.7082005810854));
#9614=CARTESIAN_POINT('',(-6.00000000000001,-2.,86.8));
#9615=CARTESIAN_POINT('Origin',(5.11429163215176E-16,-2.,86.8));
#9616=CARTESIAN_POINT('Origin',(-19.225775115544,-2.,76.0175282126611));
#9617=CARTESIAN_POINT('',(-19.225775115544,-2.,76.0175282126611));
#9618=CARTESIAN_POINT('Origin',(-6.2747399544856,-2.,83.6971563842852));
#9619=CARTESIAN_POINT('',(-6.2747399544856,-2.,83.6971563842852));
#9620=CARTESIAN_POINT('Origin',(5.11429163215176E-16,-2.,86.8));
#9621=CARTESIAN_POINT('',(-6.00000000000001,-2.,86.8));
#9622=CARTESIAN_POINT('Origin',(5.11429163215176E-16,-2.,86.8));
#9623=CARTESIAN_POINT('',(6.60407749680247,-2.,84.4791897069714));
#9624=CARTESIAN_POINT('Origin',(29.4580576969316,-2.,71.983088746998));
#9625=CARTESIAN_POINT('',(29.4580576969316,-2.,71.983088746998));
#9626=CARTESIAN_POINT('Origin',(0.29863906465954,-2.,85.678771283356));
#9627=CARTESIAN_POINT('',(23.5123684627238,-2.,63.3412203311535));
#9628=CARTESIAN_POINT('Origin',(22.0328538621538,-2.,66.4556698663697));
#9629=CARTESIAN_POINT('',(22.0328538621538,-2.,66.4556698663697));
#9630=CARTESIAN_POINT('Origin',(0.29863906465954,-2.,85.678771283356));
#9631=CARTESIAN_POINT('',(25.14540508495,-2.,70.6940477528968));
#9632=CARTESIAN_POINT('Origin',(4.87558269014984,-2.,81.777182719677));
#9633=CARTESIAN_POINT('',(4.87558269014984,-2.,81.777182719677));
#9634=CARTESIAN_POINT('Origin',(5.11429163215176E-16,-2.,86.8));
#9635=CARTESIAN_POINT('',(-4.20530738557349,-2.,81.2039844717119));
#9636=CARTESIAN_POINT('Origin',(-24.6103750011395,-2.,69.1043082562094));
#9879=UNCERTAINTY_MEASURE_WITH_UNIT(LENGTH_MEASURE(0.01),#9892,
'DISTANCE_ACCURACY_VALUE',
'Maximum model space distance between geometric entities at asserted c
onnectivities');
#9881=UNCERTAINTY_MEASURE_WITH_UNIT(LENGTH_MEASURE(0.01),#9892,
'DISTANCE_ACCURACY_VALUE',
'Maximum model space distance between geometric entities at asserted c
onnectivities');
#9889=(
GEOMETRIC_REPRESENTATION_CONTEXT(3)
GLOBAL_UNCERTAINTY_ASSIGNED_CONTEXT((#9879))
GLOBAL_UNIT_ASSIGNED_CONTEXT((#9892,#9894,#9895))
REPRESENTATION_CONTEXT('','3D')
);
#9891=(
GEOMETRIC_REPRESENTATION_CONTEXT(3)
GLOBAL_UNCERTAINTY_ASSIGNED_CONTEXT((#9881))
GLOBAL_UNIT_ASSIGNED_CONTEXT((#9892,#9894,#9895))
REPRESENTATION_CONTEXT('','3D')
);
#9892=(
LENGTH_UNIT()
NAMED_UNIT(*)
SI_UNIT(.MILLI.,.METRE.)
);
#9894=(
NAMED_UNIT(*)
PLANE_ANGLE_UNIT()
SI_UNIT($,.RADIAN.)
);
#9895=(
NAMED_UNIT(*)
SI_UNIT($,.STERADIAN.)
SOLID_ANGLE_UNIT()
);
#9903=SHAPE_DEFINITION_REPRESENTATION(#9912,#9929);
#9912=PRODUCT_DEFINITION_SHAPE('',$,#9939);
#9929=SHAPE_REPRESENTATION('',(#6182),#9889);
#9931=PRODUCT_DEFINITION_CONTEXT('part definition',#9960,'design');
#9939=PRODUCT_DEFINITION('Arm','Arm',#9948,#9931);
#9948=PRODUCT_DEFINITION_FORMATION('',$,#9969);
#9960=APPLICATION_CONTEXT(
'Core Data for Automotive Mechanical Design Process');
#9961=PRODUCT_CONTEXT('part definition',#9960,'mechanical');
#9969=PRODUCT('Arm','Arm',$,(#9961));
#9975=PRESENTATION_STYLE_ASSIGNMENT((#9980));
#9980=SURFACE_STYLE_USAGE(.BOTH.,#9985);
#9985=SURFACE_SIDE_STYLE('',(#9990));
#9990=SURFACE_STYLE_FILL_AREA(#9995);
#9995=FILL_AREA_STYLE('Opaque(203,203,203)',(#10000));
#10000=FILL_AREA_STYLE_COLOUR('Opaque(203,203,203)',#10005);
#10005=COLOUR_RGB('Opaque(203,203,203)', 0.40784314, 0.44705882, 0.49803922);
ENDSEC;
END-ISO-10303-21;
